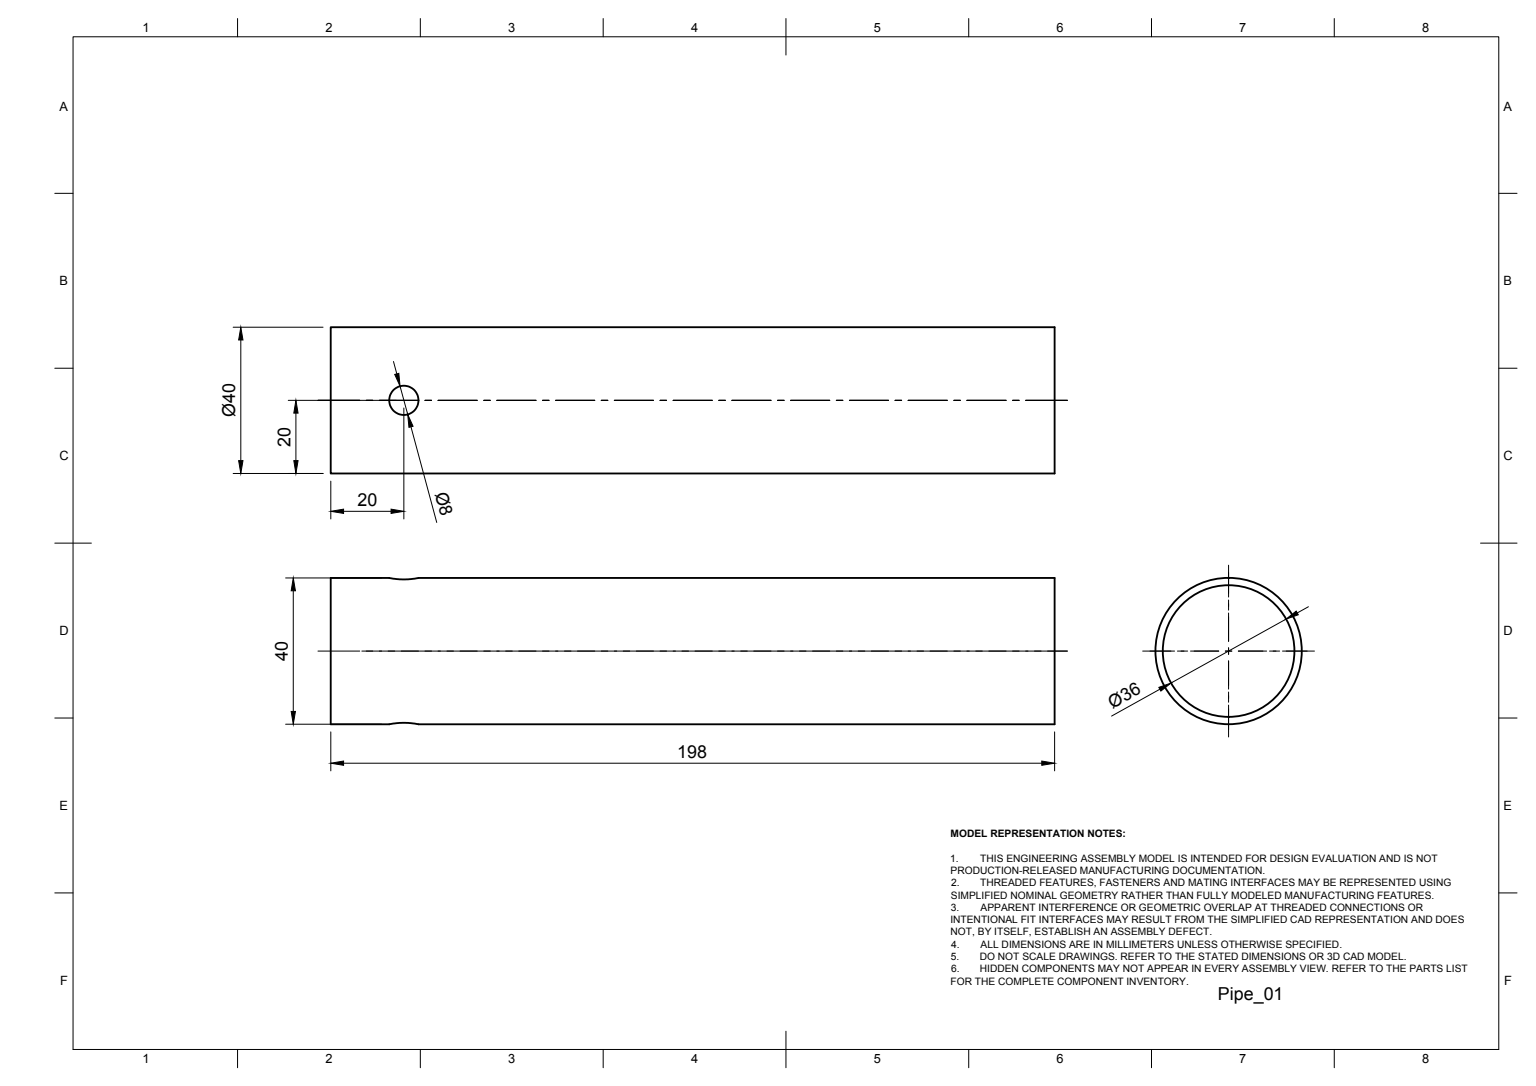
ISO-10303-21;
HEADER;
/* Generated by software containing ST-Developer
 * from STEP Tools, Inc. (www.steptools.com) 
 */

FILE_DESCRIPTION(
/* description */ (''),
/* implementation_level */ '2;1');

FILE_NAME(
/* name */ 'Pipe_01.step',
/* time_stamp */ '2026-10-06T13:31:15-07:00',
/* author */ (''),
/* organization */ (''),
/* preprocessor_version */ 'ST-DEVELOPER v20.2',
/* originating_system */ 'Autodesk Translation Framework v15.15.0.0',
/* authorisation */ '');

FILE_SCHEMA (('AUTOMOTIVE_DESIGN { 1 0 10303 214 3 1 1 }'));
ENDSEC;

DATA;
#10=MECHANICAL_DESIGN_GEOMETRIC_PRESENTATION_REPRESENTATION('',(#79),#3154);
#61=SHAPE_REPRESENTATION_RELATIONSHIP('SRR','None',#3189,#70);
#70=ADVANCED_BREP_SHAPE_REPRESENTATION('',(#88),#3145);
#79=STYLED_ITEM('',(#3243),#88);
#88=MANIFOLD_SOLID_BREP('Body1',#1081);
#97=PLANE('',#1200);
#98=PLANE('',#1201);
#128=FACE_BOUND('',#233,.T.);
#129=FACE_BOUND('',#235,.T.);
#130=FACE_BOUND('',#237,.T.);
#131=FACE_BOUND('',#239,.T.);
#139=CIRCLE('',#1195,18.);
#140=CIRCLE('',#1196,18.);
#141=CIRCLE('',#1198,20.);
#142=CIRCLE('',#1199,20.);
#171=FACE_OUTER_BOUND('',#230,.T.);
#172=FACE_OUTER_BOUND('',#231,.T.);
#173=FACE_OUTER_BOUND('',#232,.T.);
#174=FACE_OUTER_BOUND('',#234,.T.);
#175=FACE_OUTER_BOUND('',#236,.T.);
#176=FACE_OUTER_BOUND('',#238,.T.);
#230=EDGE_LOOP('',(#720,#721,#722,#723,#724,#725,#726,#727));
#231=EDGE_LOOP('',(#728,#729,#730,#731,#732,#733));
#232=EDGE_LOOP('',(#734,#735,#736,#737,#738,#739,#740,#741,#742));
#233=EDGE_LOOP('',(#743,#744));
#234=EDGE_LOOP('',(#745,#746,#747,#748,#749,#750,#751,#752,#753));
#235=EDGE_LOOP('',(#754,#755));
#236=EDGE_LOOP('',(#756));
#237=EDGE_LOOP('',(#757));
#238=EDGE_LOOP('',(#758));
#239=EDGE_LOOP('',(#759));
#300=LINE('',#1580,#366);
#301=LINE('',#1672,#367);
#302=LINE('',#1713,#368);
#303=LINE('',#1715,#369);
#304=LINE('',#1720,#370);
#305=LINE('',#1722,#371);
#366=VECTOR('',#1292,3.99999999999999);
#367=VECTOR('',#1295,3.99999999999999);
#368=VECTOR('',#1300,18.);
#369=VECTOR('',#1301,18.);
#370=VECTOR('',#1308,20.);
#371=VECTOR('',#1309,20.);
#432=B_SPLINE_CURVE_WITH_KNOTS('',3,(#1549,#1550,#1551,#1552,#1553,#1554,
#1555,#1556,#1557,#1558,#1559,#1560,#1561,#1562,#1563,#1564,#1565,#1566,
#1567),.UNSPECIFIED.,.F.,.F.,(4,2,2,2,3,2,2,2,4),(-0.604455473723513,-0.453345839217834,
-0.302236204712155,-0.151118102356077,0.,0.151118102356077,0.302236204712155,
0.453345839217834,0.604455473723513),.UNSPECIFIED.);
#433=B_SPLINE_CURVE_WITH_KNOTS('',3,(#1569,#1570,#1571,#1572,#1573,#1574,
#1575,#1576,#1577,#1578),.UNSPECIFIED.,.F.,.F.,(4,2,2,2,4),(-1.81336642117054,
-1.66225678666486,-1.51114715215918,-1.3600290498031,-1.20891094744703),
 .UNSPECIFIED.);
#434=B_SPLINE_CURVE_WITH_KNOTS('',3,(#1582,#1583,#1584,#1585,#1586,#1587,
#1588,#1589,#1590,#1591),.UNSPECIFIED.,.F.,.F.,(4,2,2,2,4),(1.20975547030872,
1.36098142054494,1.51220737078115,1.66342028812212,1.81463320546308),
 .UNSPECIFIED.);
#435=B_SPLINE_CURVE_WITH_KNOTS('',3,(#1593,#1594,#1595,#1596,#1597,#1598,
#1599,#1600,#1601,#1602,#1603,#1604,#1605,#1606,#1607,#1608,#1609,#1610,
#1611),.UNSPECIFIED.,.F.,.F.,(4,2,2,2,3,2,2,2,4),(1.81463320546308,1.96584612280404,
2.11705904014501,2.26828499038122,2.41951094061744,2.57073689085366,2.72196284108987,
2.87317575843084,3.0243886757718),.UNSPECIFIED.);
#436=B_SPLINE_CURVE_WITH_KNOTS('',3,(#1612,#1613,#1614,#1615,#1616,#1617,
#1618,#1619,#1620,#1621),.UNSPECIFIED.,.F.,.F.,(4,2,2,2,4),(0.60487773515436,
0.756090652495323,0.907303569836285,1.0585295200725,1.20975547030872),
 .UNSPECIFIED.);
#437=B_SPLINE_CURVE_WITH_KNOTS('',3,(#1622,#1623,#1624,#1625,#1626,#1627,
#1628,#1629,#1630,#1631),.UNSPECIFIED.,.F.,.F.,(4,2,2,2,4),(-1.20891094744703,
-1.05779284509095,-0.906674742734871,-0.755565108229192,-0.604455473723513),
 .UNSPECIFIED.);
#438=B_SPLINE_CURVE_WITH_KNOTS('',3,(#1635,#1636,#1637,#1638,#1639,#1640,
#1641,#1642,#1643,#1644,#1645,#1646,#1647,#1648,#1649,#1650,#1651,#1652),
 .UNSPECIFIED.,.F.,.F.,(4,2,2,2,2,2,2,2,4),(-2.41951094061744,-2.26828499038122,
-2.11705904014501,-1.96584612280404,-1.81463320546308,-1.66342028812212,
-1.51220737078115,-1.36098142054494,-1.20975547030872),.UNSPECIFIED.);
#439=B_SPLINE_CURVE_WITH_KNOTS('',3,(#1653,#1654,#1655,#1656,#1657,#1658,
#1659,#1660,#1661,#1662,#1663,#1664,#1665,#1666,#1667,#1668,#1669,#1670),
 .UNSPECIFIED.,.F.,.F.,(4,2,2,2,2,2,2,2,4),(-1.20975547030872,-1.0585295200725,
-0.907303569836286,-0.756090652495323,-0.60487773515436,-0.453664817813397,
-0.302451900472434,-0.151225950236217,0.),.UNSPECIFIED.);
#440=B_SPLINE_CURVE_WITH_KNOTS('',3,(#1674,#1675,#1676,#1677,#1678,#1679,
#1680,#1681,#1682,#1683,#1684,#1685,#1686,#1687,#1688,#1689,#1690,#1691),
 .UNSPECIFIED.,.F.,.F.,(4,2,2,2,2,2,2,2,4),(0.,0.151118102356077,0.302236204712155,
0.453345839217834,0.604455473723513,0.755565108229192,0.906674742734871,
1.05779284509095,1.20891094744703),.UNSPECIFIED.);
#441=B_SPLINE_CURVE_WITH_KNOTS('',3,(#1692,#1693,#1694,#1695,#1696,#1697,
#1698,#1699,#1700,#1701,#1702,#1703,#1704,#1705,#1706,#1707,#1708,#1709),
 .UNSPECIFIED.,.F.,.F.,(4,2,2,2,2,2,2,2,4),(1.20891094744703,1.3600290498031,
1.51114715215918,1.66225678666486,1.81336642117054,1.96447605567622,2.1155856901819,
2.26670379253797,2.41782189489405),.UNSPECIFIED.);
#478=VERTEX_POINT('',#1547);
#479=VERTEX_POINT('',#1548);
#480=VERTEX_POINT('',#1568);
#481=VERTEX_POINT('',#1579);
#482=VERTEX_POINT('',#1581);
#483=VERTEX_POINT('',#1592);
#484=VERTEX_POINT('',#1633);
#485=VERTEX_POINT('',#1634);
#486=VERTEX_POINT('',#1671);
#487=VERTEX_POINT('',#1673);
#488=VERTEX_POINT('',#1711);
#489=VERTEX_POINT('',#1714);
#490=VERTEX_POINT('',#1718);
#491=VERTEX_POINT('',#1721);
#576=EDGE_CURVE('',#478,#479,#432,.F.);
#577=EDGE_CURVE('',#480,#478,#433,.F.);
#578=EDGE_CURVE('',#480,#481,#300,.T.);
#579=EDGE_CURVE('',#482,#481,#434,.F.);
#580=EDGE_CURVE('',#483,#482,#435,.F.);
#581=EDGE_CURVE('',#481,#483,#436,.F.);
#582=EDGE_CURVE('',#479,#480,#437,.F.);
#583=EDGE_CURVE('',#484,#485,#438,.T.);
#584=EDGE_CURVE('',#485,#484,#439,.T.);
#585=EDGE_CURVE('',#485,#486,#301,.T.);
#586=EDGE_CURVE('',#487,#486,#440,.T.);
#587=EDGE_CURVE('',#486,#487,#441,.T.);
#588=EDGE_CURVE('',#488,#488,#139,.T.);
#589=EDGE_CURVE('',#488,#482,#302,.T.);
#590=EDGE_CURVE('',#483,#489,#303,.T.);
#591=EDGE_CURVE('',#489,#489,#140,.T.);
#592=EDGE_CURVE('',#490,#490,#141,.T.);
#593=EDGE_CURVE('',#490,#479,#304,.T.);
#594=EDGE_CURVE('',#478,#491,#305,.T.);
#595=EDGE_CURVE('',#491,#491,#142,.T.);
#720=ORIENTED_EDGE('',*,*,#576,.F.);
#721=ORIENTED_EDGE('',*,*,#577,.F.);
#722=ORIENTED_EDGE('',*,*,#578,.T.);
#723=ORIENTED_EDGE('',*,*,#579,.F.);
#724=ORIENTED_EDGE('',*,*,#580,.F.);
#725=ORIENTED_EDGE('',*,*,#581,.F.);
#726=ORIENTED_EDGE('',*,*,#578,.F.);
#727=ORIENTED_EDGE('',*,*,#582,.F.);
#728=ORIENTED_EDGE('',*,*,#583,.F.);
#729=ORIENTED_EDGE('',*,*,#584,.F.);
#730=ORIENTED_EDGE('',*,*,#585,.T.);
#731=ORIENTED_EDGE('',*,*,#586,.F.);
#732=ORIENTED_EDGE('',*,*,#587,.F.);
#733=ORIENTED_EDGE('',*,*,#585,.F.);
#734=ORIENTED_EDGE('',*,*,#588,.T.);
#735=ORIENTED_EDGE('',*,*,#589,.T.);
#736=ORIENTED_EDGE('',*,*,#579,.T.);
#737=ORIENTED_EDGE('',*,*,#581,.T.);
#738=ORIENTED_EDGE('',*,*,#590,.T.);
#739=ORIENTED_EDGE('',*,*,#591,.F.);
#740=ORIENTED_EDGE('',*,*,#590,.F.);
#741=ORIENTED_EDGE('',*,*,#580,.T.);
#742=ORIENTED_EDGE('',*,*,#589,.F.);
#743=ORIENTED_EDGE('',*,*,#583,.T.);
#744=ORIENTED_EDGE('',*,*,#584,.T.);
#745=ORIENTED_EDGE('',*,*,#592,.F.);
#746=ORIENTED_EDGE('',*,*,#593,.T.);
#747=ORIENTED_EDGE('',*,*,#582,.T.);
#748=ORIENTED_EDGE('',*,*,#577,.T.);
#749=ORIENTED_EDGE('',*,*,#594,.T.);
#750=ORIENTED_EDGE('',*,*,#595,.T.);
#751=ORIENTED_EDGE('',*,*,#594,.F.);
#752=ORIENTED_EDGE('',*,*,#576,.T.);
#753=ORIENTED_EDGE('',*,*,#593,.F.);
#754=ORIENTED_EDGE('',*,*,#586,.T.);
#755=ORIENTED_EDGE('',*,*,#587,.T.);
#756=ORIENTED_EDGE('',*,*,#592,.T.);
#757=ORIENTED_EDGE('',*,*,#591,.T.);
#758=ORIENTED_EDGE('',*,*,#595,.F.);
#759=ORIENTED_EDGE('',*,*,#588,.F.);
#1008=CYLINDRICAL_SURFACE('',#1192,3.99999999999999);
#1009=CYLINDRICAL_SURFACE('',#1193,3.99999999999999);
#1010=CYLINDRICAL_SURFACE('',#1194,18.);
#1011=CYLINDRICAL_SURFACE('',#1197,20.);
#1022=ADVANCED_FACE('',(#171),#1008,.F.);
#1023=ADVANCED_FACE('',(#172),#1009,.F.);
#1024=ADVANCED_FACE('',(#173,#128),#1010,.F.);
#1025=ADVANCED_FACE('',(#174,#129),#1011,.T.);
#1026=ADVANCED_FACE('',(#175,#130),#97,.T.);
#1027=ADVANCED_FACE('',(#176,#131),#98,.F.);
#1081=CLOSED_SHELL('',(#1022,#1023,#1024,#1025,#1026,#1027));
#1191=AXIS2_PLACEMENT_3D('',#1545,#1288,#1289);
#1192=AXIS2_PLACEMENT_3D('',#1546,#1290,#1291);
#1193=AXIS2_PLACEMENT_3D('',#1632,#1293,#1294);
#1194=AXIS2_PLACEMENT_3D('',#1710,#1296,#1297);
#1195=AXIS2_PLACEMENT_3D('',#1712,#1298,#1299);
#1196=AXIS2_PLACEMENT_3D('',#1716,#1302,#1303);
#1197=AXIS2_PLACEMENT_3D('',#1717,#1304,#1305);
#1198=AXIS2_PLACEMENT_3D('',#1719,#1306,#1307);
#1199=AXIS2_PLACEMENT_3D('',#1723,#1310,#1311);
#1200=AXIS2_PLACEMENT_3D('',#1724,#1312,#1313);
#1201=AXIS2_PLACEMENT_3D('',#1725,#1314,#1315);
#1288=DIRECTION('axis',(0.,0.,1.));
#1289=DIRECTION('refdir',(1.,0.,0.));
#1290=DIRECTION('center_axis',(1.,0.,0.));
#1291=DIRECTION('ref_axis',(0.,1.,0.));
#1292=DIRECTION('',(1.,0.,0.));
#1293=DIRECTION('center_axis',(1.,0.,0.));
#1294=DIRECTION('ref_axis',(0.,1.,0.));
#1295=DIRECTION('',(1.,0.,0.));
#1296=DIRECTION('center_axis',(0.,0.,1.));
#1297=DIRECTION('ref_axis',(1.,0.,0.));
#1298=DIRECTION('center_axis',(0.,0.,-1.));
#1299=DIRECTION('ref_axis',(1.,0.,0.));
#1300=DIRECTION('',(0.,0.,1.));
#1301=DIRECTION('',(0.,0.,1.));
#1302=DIRECTION('center_axis',(0.,0.,-1.));
#1303=DIRECTION('ref_axis',(1.,0.,0.));
#1304=DIRECTION('center_axis',(0.,0.,1.));
#1305=DIRECTION('ref_axis',(1.,0.,0.));
#1306=DIRECTION('center_axis',(0.,0.,1.));
#1307=DIRECTION('ref_axis',(1.,0.,0.));
#1308=DIRECTION('',(0.,0.,-1.));
#1309=DIRECTION('',(0.,0.,-1.));
#1310=DIRECTION('center_axis',(0.,0.,1.));
#1311=DIRECTION('ref_axis',(1.,0.,0.));
#1312=DIRECTION('center_axis',(0.,0.,1.));
#1313=DIRECTION('ref_axis',(1.,0.,0.));
#1314=DIRECTION('center_axis',(0.,0.,1.));
#1315=DIRECTION('ref_axis',(1.,0.,0.));
#1545=CARTESIAN_POINT('',(0.,0.,0.));
#1546=CARTESIAN_POINT('Origin',(0.,0.,180.));
#1547=CARTESIAN_POINT('',(-20.,-1.98792512857715E-15,176.));
#1548=CARTESIAN_POINT('',(-20.,-1.05117445154967E-15,184.));
#1549=CARTESIAN_POINT('Ctrl Pts',(-20.,-2.77555756156289E-16,184.));
#1550=CARTESIAN_POINT('Ctrl Pts',(-20.,0.503698781685596,184.));
#1551=CARTESIAN_POINT('Ctrl Pts',(-19.9790475458833,1.04005322432747,183.899058168943));
#1552=CARTESIAN_POINT('Ctrl Pts',(-19.9033338860745,2.02517944479051,183.490417366179));
#1553=CARTESIAN_POINT('Ctrl Pts',(-19.8496135055327,2.47406169858037,183.182792550912));
#1554=CARTESIAN_POINT('Ctrl Pts',(-19.7483634040773,3.18281240876835,182.474041840724));
#1555=CARTESIAN_POINT('Ctrl Pts',(-19.6941660317108,3.4904216705935,182.02516802012));
#1556=CARTESIAN_POINT('Ctrl Pts',(-19.6173550647379,3.89905118499443,181.040071108648));
#1557=CARTESIAN_POINT('Ctrl Pts',(-19.5959179422654,3.99999999999999,180.503727007854));
#1558=CARTESIAN_POINT('Ctrl Pts',(-19.5959179422654,3.99999999999999,180.));
#1559=CARTESIAN_POINT('Ctrl Pts',(-19.5959179422654,3.99999999999999,179.496272992146));
#1560=CARTESIAN_POINT('Ctrl Pts',(-19.6173550647379,3.89905118499443,178.959928891352));
#1561=CARTESIAN_POINT('Ctrl Pts',(-19.6941660317108,3.4904216705935,177.97483197988));
#1562=CARTESIAN_POINT('Ctrl Pts',(-19.7483634040773,3.18281240876835,177.525958159276));
#1563=CARTESIAN_POINT('Ctrl Pts',(-19.8496135055327,2.47406169858037,176.817207449088));
#1564=CARTESIAN_POINT('Ctrl Pts',(-19.9033338860745,2.02517944479051,176.509582633821));
#1565=CARTESIAN_POINT('Ctrl Pts',(-19.9790475458833,1.04005322432747,176.100941831057));
#1566=CARTESIAN_POINT('Ctrl Pts',(-20.,0.503698781685596,176.));
#1567=CARTESIAN_POINT('Ctrl Pts',(-20.,-1.2490009027033E-15,176.));
#1568=CARTESIAN_POINT('',(-19.5959179422654,-3.99999999999999,180.));
#1569=CARTESIAN_POINT('Ctrl Pts',(-20.,-9.71445146547012E-16,176.));
#1570=CARTESIAN_POINT('Ctrl Pts',(-20.,-0.503698781685598,176.));
#1571=CARTESIAN_POINT('Ctrl Pts',(-19.9790475458833,-1.04005322432746,176.100941831057));
#1572=CARTESIAN_POINT('Ctrl Pts',(-19.9033338860745,-2.0251794447905,176.509582633821));
#1573=CARTESIAN_POINT('Ctrl Pts',(-19.8496135055327,-2.47406169858037,176.817207449088));
#1574=CARTESIAN_POINT('Ctrl Pts',(-19.7483634040773,-3.18281240876835,177.525958159276));
#1575=CARTESIAN_POINT('Ctrl Pts',(-19.6941660317108,-3.4904216705935,177.97483197988));
#1576=CARTESIAN_POINT('Ctrl Pts',(-19.6173550647379,-3.89905118499443,178.959928891352));
#1577=CARTESIAN_POINT('Ctrl Pts',(-19.5959179422654,-3.99999999999999,179.496272992146));
#1578=CARTESIAN_POINT('Ctrl Pts',(-19.5959179422654,-3.99999999999999,180.));
#1579=CARTESIAN_POINT('',(-17.5499287747842,-3.99999999999999,180.));
#1580=CARTESIAN_POINT('',(0.,-3.99999999999999,180.));
#1581=CARTESIAN_POINT('',(-18.,-2.48996090001406E-15,176.));
#1582=CARTESIAN_POINT('Ctrl Pts',(-17.5499287747842,-3.99999999999999,180.));
#1583=CARTESIAN_POINT('Ctrl Pts',(-17.5499287747842,-3.99999999999999,179.495913499213));
#1584=CARTESIAN_POINT('Ctrl Pts',(-17.5739034455062,-3.89891257329756,178.959425202916));
#1585=CARTESIAN_POINT('Ctrl Pts',(-17.6596205619409,-3.49018656101197,177.97443488127));
#1586=CARTESIAN_POINT('Ctrl Pts',(-17.7200302505161,-3.18263533348267,177.52578108399));
#1587=CARTESIAN_POINT('Ctrl Pts',(-17.8327425616729,-2.47424944224197,176.81739519275));
#1588=CARTESIAN_POINT('Ctrl Pts',(-17.8924945311419,-2.02558278587652,176.509820096788));
#1589=CARTESIAN_POINT('Ctrl Pts',(-17.9766962279685,-1.04054739507664,176.101076729386));
#1590=CARTESIAN_POINT('Ctrl Pts',(-18.,-0.504043057803209,176.));
#1591=CARTESIAN_POINT('Ctrl Pts',(-18.,9.71445146547012E-16,176.));
#1592=CARTESIAN_POINT('',(-18.,-2.28179408289685E-15,184.));
#1593=CARTESIAN_POINT('Ctrl Pts',(-18.,-2.77555756156289E-15,176.));
#1594=CARTESIAN_POINT('Ctrl Pts',(-18.,0.504043057803207,176.));
#1595=CARTESIAN_POINT('Ctrl Pts',(-17.9766962279685,1.04054739507664,176.101076729386));
#1596=CARTESIAN_POINT('Ctrl Pts',(-17.8924945311419,2.02558278587652,176.509820096788));
#1597=CARTESIAN_POINT('Ctrl Pts',(-17.8327425616729,2.47424944224197,176.81739519275));
#1598=CARTESIAN_POINT('Ctrl Pts',(-17.7200302505161,3.18263533348267,177.52578108399));
#1599=CARTESIAN_POINT('Ctrl Pts',(-17.6596205619409,3.49018656101197,177.97443488127));
#1600=CARTESIAN_POINT('Ctrl Pts',(-17.5739034455062,3.89891257329756,178.959425202916));
#1601=CARTESIAN_POINT('Ctrl Pts',(-17.5499287747842,3.99999999999999,179.495913499213));
#1602=CARTESIAN_POINT('Ctrl Pts',(-17.5499287747842,3.99999999999999,180.));
#1603=CARTESIAN_POINT('Ctrl Pts',(-17.5499287747842,3.99999999999999,180.504086500787));
#1604=CARTESIAN_POINT('Ctrl Pts',(-17.5739034455062,3.89891257329756,181.040574797084));
#1605=CARTESIAN_POINT('Ctrl Pts',(-17.6596205619409,3.49018656101197,182.02556511873));
#1606=CARTESIAN_POINT('Ctrl Pts',(-17.7200302505161,3.18263533348267,182.47421891601));
#1607=CARTESIAN_POINT('Ctrl Pts',(-17.8327425616729,2.47424944224197,183.18260480725));
#1608=CARTESIAN_POINT('Ctrl Pts',(-17.8924945311419,2.02558278587652,183.490179903212));
#1609=CARTESIAN_POINT('Ctrl Pts',(-17.9766962279685,1.04054739507664,183.898923270614));
#1610=CARTESIAN_POINT('Ctrl Pts',(-18.,0.50404305780321,184.));
#1611=CARTESIAN_POINT('Ctrl Pts',(-18.,6.93889390390723E-16,184.));
#1612=CARTESIAN_POINT('Ctrl Pts',(-18.,7.63278329429795E-16,184.));
#1613=CARTESIAN_POINT('Ctrl Pts',(-18.,-0.504043057803209,184.));
#1614=CARTESIAN_POINT('Ctrl Pts',(-17.9766962279685,-1.04054739507664,183.898923270614));
#1615=CARTESIAN_POINT('Ctrl Pts',(-17.8924945311419,-2.02558278587652,183.490179903212));
#1616=CARTESIAN_POINT('Ctrl Pts',(-17.8327425616729,-2.47424944224197,183.18260480725));
#1617=CARTESIAN_POINT('Ctrl Pts',(-17.7200302505161,-3.18263533348267,182.47421891601));
#1618=CARTESIAN_POINT('Ctrl Pts',(-17.6596205619409,-3.49018656101197,182.02556511873));
#1619=CARTESIAN_POINT('Ctrl Pts',(-17.5739034455062,-3.89891257329756,181.040574797084));
#1620=CARTESIAN_POINT('Ctrl Pts',(-17.5499287747842,-3.99999999999999,180.504086500787));
#1621=CARTESIAN_POINT('Ctrl Pts',(-17.5499287747842,-3.99999999999999,180.));
#1622=CARTESIAN_POINT('Ctrl Pts',(-19.5959179422654,-3.99999999999999,180.));
#1623=CARTESIAN_POINT('Ctrl Pts',(-19.5959179422654,-3.99999999999999,180.503727007854));
#1624=CARTESIAN_POINT('Ctrl Pts',(-19.6173550647379,-3.89905118499443,181.040071108648));
#1625=CARTESIAN_POINT('Ctrl Pts',(-19.6941660317108,-3.4904216705935,182.02516802012));
#1626=CARTESIAN_POINT('Ctrl Pts',(-19.7483634040773,-3.18281240876835,182.474041840724));
#1627=CARTESIAN_POINT('Ctrl Pts',(-19.8496135055327,-2.47406169858037,183.182792550912));
#1628=CARTESIAN_POINT('Ctrl Pts',(-19.9033338860745,-2.02517944479051,183.490417366179));
#1629=CARTESIAN_POINT('Ctrl Pts',(-19.9790475458833,-1.04005322432747,183.899058168943));
#1630=CARTESIAN_POINT('Ctrl Pts',(-20.,-0.503698781685596,184.));
#1631=CARTESIAN_POINT('Ctrl Pts',(-20.,3.46944695195361E-16,184.));
#1632=CARTESIAN_POINT('Origin',(0.,0.,180.));
#1633=CARTESIAN_POINT('',(17.5499287747842,3.99999999999999,180.));
#1634=CARTESIAN_POINT('',(17.5499287747842,-3.99999999999999,180.));
#1635=CARTESIAN_POINT('Ctrl Pts',(17.5499287747842,3.99999999999999,180.));
#1636=CARTESIAN_POINT('Ctrl Pts',(17.5499287747842,3.99999999999999,180.504086500787));
#1637=CARTESIAN_POINT('Ctrl Pts',(17.5739034455062,3.89891257329756,181.040574797084));
#1638=CARTESIAN_POINT('Ctrl Pts',(17.6596205619409,3.49018656101197,182.02556511873));
#1639=CARTESIAN_POINT('Ctrl Pts',(17.7200302505161,3.18263533348267,182.47421891601));
#1640=CARTESIAN_POINT('Ctrl Pts',(17.8327425616729,2.47424944224197,183.18260480725));
#1641=CARTESIAN_POINT('Ctrl Pts',(17.8924945311419,2.0255827858765,183.490179903212));
#1642=CARTESIAN_POINT('Ctrl Pts',(17.9766962279685,1.04054739507661,183.898923270614));
#1643=CARTESIAN_POINT('Ctrl Pts',(18.,0.50404305780321,184.));
#1644=CARTESIAN_POINT('Ctrl Pts',(18.,-0.504043057803209,184.));
#1645=CARTESIAN_POINT('Ctrl Pts',(17.9766962279685,-1.04054739507664,183.898923270614));
#1646=CARTESIAN_POINT('Ctrl Pts',(17.8924945311419,-2.02558278587652,183.490179903212));
#1647=CARTESIAN_POINT('Ctrl Pts',(17.8327425616729,-2.47424944224197,183.18260480725));
#1648=CARTESIAN_POINT('Ctrl Pts',(17.7200302505161,-3.18263533348267,182.47421891601));
#1649=CARTESIAN_POINT('Ctrl Pts',(17.6596205619409,-3.49018656101197,182.02556511873));
#1650=CARTESIAN_POINT('Ctrl Pts',(17.5739034455062,-3.89891257329756,181.040574797084));
#1651=CARTESIAN_POINT('Ctrl Pts',(17.5499287747842,-3.99999999999999,180.504086500787));
#1652=CARTESIAN_POINT('Ctrl Pts',(17.5499287747842,-3.99999999999999,180.));
#1653=CARTESIAN_POINT('Ctrl Pts',(17.5499287747842,-3.99999999999999,180.));
#1654=CARTESIAN_POINT('Ctrl Pts',(17.5499287747842,-3.99999999999999,179.495913499213));
#1655=CARTESIAN_POINT('Ctrl Pts',(17.5739034455062,-3.89891257329756,178.959425202916));
#1656=CARTESIAN_POINT('Ctrl Pts',(17.6596205619409,-3.49018656101197,177.97443488127));
#1657=CARTESIAN_POINT('Ctrl Pts',(17.7200302505161,-3.18263533348267,177.52578108399));
#1658=CARTESIAN_POINT('Ctrl Pts',(17.8327425616729,-2.47424944224197,176.81739519275));
#1659=CARTESIAN_POINT('Ctrl Pts',(17.8924945311419,-2.02558278587652,176.509820096788));
#1660=CARTESIAN_POINT('Ctrl Pts',(17.9766962279685,-1.04054739507664,176.101076729386));
#1661=CARTESIAN_POINT('Ctrl Pts',(18.,-0.50404305780321,176.));
#1662=CARTESIAN_POINT('Ctrl Pts',(18.,0.504043057803209,176.));
#1663=CARTESIAN_POINT('Ctrl Pts',(17.9766962279685,1.04054739507664,176.101076729386));
#1664=CARTESIAN_POINT('Ctrl Pts',(17.8924945311419,2.02558278587652,176.509820096788));
#1665=CARTESIAN_POINT('Ctrl Pts',(17.8327425616729,2.47424944224197,176.81739519275));
#1666=CARTESIAN_POINT('Ctrl Pts',(17.7200302505161,3.18263533348267,177.52578108399));
#1667=CARTESIAN_POINT('Ctrl Pts',(17.6596205619409,3.49018656101197,177.97443488127));
#1668=CARTESIAN_POINT('Ctrl Pts',(17.5739034455062,3.89891257329756,178.959425202916));
#1669=CARTESIAN_POINT('Ctrl Pts',(17.5499287747842,3.99999999999999,179.495913499213));
#1670=CARTESIAN_POINT('Ctrl Pts',(17.5499287747842,3.99999999999999,180.));
#1671=CARTESIAN_POINT('',(19.5959179422654,-3.99999999999999,180.));
#1672=CARTESIAN_POINT('',(0.,-3.99999999999999,180.));
#1673=CARTESIAN_POINT('',(19.5959179422654,3.99999999999999,180.));
#1674=CARTESIAN_POINT('Ctrl Pts',(19.5959179422654,3.99999999999999,180.));
#1675=CARTESIAN_POINT('Ctrl Pts',(19.5959179422654,3.99999999999999,179.496272992146));
#1676=CARTESIAN_POINT('Ctrl Pts',(19.6173550647379,3.89905118499443,178.959928891352));
#1677=CARTESIAN_POINT('Ctrl Pts',(19.6941660317108,3.4904216705935,177.97483197988));
#1678=CARTESIAN_POINT('Ctrl Pts',(19.7483634040773,3.18281240876835,177.525958159276));
#1679=CARTESIAN_POINT('Ctrl Pts',(19.8496135055327,2.47406169858037,176.817207449088));
#1680=CARTESIAN_POINT('Ctrl Pts',(19.9033338860745,2.02517944479051,176.509582633821));
#1681=CARTESIAN_POINT('Ctrl Pts',(19.9790475458833,1.04005322432747,176.100941831057));
#1682=CARTESIAN_POINT('Ctrl Pts',(20.,0.503698781685596,176.));
#1683=CARTESIAN_POINT('Ctrl Pts',(20.,-0.503698781685597,176.));
#1684=CARTESIAN_POINT('Ctrl Pts',(19.9790475458833,-1.04005322432747,176.100941831057));
#1685=CARTESIAN_POINT('Ctrl Pts',(19.9033338860745,-2.02517944479051,176.509582633821));
#1686=CARTESIAN_POINT('Ctrl Pts',(19.8496135055327,-2.47406169858037,176.817207449088));
#1687=CARTESIAN_POINT('Ctrl Pts',(19.7483634040773,-3.18281240876835,177.525958159276));
#1688=CARTESIAN_POINT('Ctrl Pts',(19.6941660317108,-3.4904216705935,177.97483197988));
#1689=CARTESIAN_POINT('Ctrl Pts',(19.6173550647379,-3.89905118499443,178.959928891352));
#1690=CARTESIAN_POINT('Ctrl Pts',(19.5959179422654,-3.99999999999999,179.496272992146));
#1691=CARTESIAN_POINT('Ctrl Pts',(19.5959179422654,-3.99999999999999,180.));
#1692=CARTESIAN_POINT('Ctrl Pts',(19.5959179422654,-3.99999999999999,180.));
#1693=CARTESIAN_POINT('Ctrl Pts',(19.5959179422654,-3.99999999999999,180.503727007854));
#1694=CARTESIAN_POINT('Ctrl Pts',(19.6173550647379,-3.89905118499443,181.040071108648));
#1695=CARTESIAN_POINT('Ctrl Pts',(19.6941660317108,-3.49042167059349,182.02516802012));
#1696=CARTESIAN_POINT('Ctrl Pts',(19.7483634040773,-3.18281240876835,182.474041840724));
#1697=CARTESIAN_POINT('Ctrl Pts',(19.8496135055327,-2.47406169858037,183.182792550912));
#1698=CARTESIAN_POINT('Ctrl Pts',(19.9033338860745,-2.02517944479048,183.490417366179));
#1699=CARTESIAN_POINT('Ctrl Pts',(19.9790475458833,-1.04005322432745,183.899058168943));
#1700=CARTESIAN_POINT('Ctrl Pts',(20.,-0.503698781685597,184.));
#1701=CARTESIAN_POINT('Ctrl Pts',(20.,0.503698781685597,184.));
#1702=CARTESIAN_POINT('Ctrl Pts',(19.9790475458833,1.04005322432747,183.899058168943));
#1703=CARTESIAN_POINT('Ctrl Pts',(19.9033338860745,2.02517944479051,183.490417366179));
#1704=CARTESIAN_POINT('Ctrl Pts',(19.8496135055327,2.47406169858037,183.182792550912));
#1705=CARTESIAN_POINT('Ctrl Pts',(19.7483634040773,3.18281240876835,182.474041840724));
#1706=CARTESIAN_POINT('Ctrl Pts',(19.6941660317108,3.4904216705935,182.02516802012));
#1707=CARTESIAN_POINT('Ctrl Pts',(19.6173550647379,3.89905118499443,181.040071108648));
#1708=CARTESIAN_POINT('Ctrl Pts',(19.5959179422654,3.99999999999999,180.503727007854));
#1709=CARTESIAN_POINT('Ctrl Pts',(19.5959179422654,3.99999999999999,180.));
#1710=CARTESIAN_POINT('Origin',(0.,0.,0.));
#1711=CARTESIAN_POINT('',(-18.,2.20436423846524E-15,2.));
#1712=CARTESIAN_POINT('Origin',(0.,0.,2.));
#1713=CARTESIAN_POINT('',(-18.,-2.20436423846524E-15,0.));
#1714=CARTESIAN_POINT('',(-18.,-2.20436423846524E-15,200.));
#1715=CARTESIAN_POINT('',(-18.,-2.20436423846524E-15,0.));
#1716=CARTESIAN_POINT('Origin',(0.,0.,200.));
#1717=CARTESIAN_POINT('Origin',(0.,0.,0.));
#1718=CARTESIAN_POINT('',(-20.,-2.44929359829471E-15,200.));
#1719=CARTESIAN_POINT('Origin',(0.,0.,200.));
#1720=CARTESIAN_POINT('',(-20.,-2.44929359829471E-15,0.));
#1721=CARTESIAN_POINT('',(-20.,-2.44929359829471E-15,2.));
#1722=CARTESIAN_POINT('',(-20.,-2.44929359829471E-15,0.));
#1723=CARTESIAN_POINT('Origin',(0.,0.,2.));
#1724=CARTESIAN_POINT('Origin',(0.,0.,200.));
#1725=CARTESIAN_POINT('Origin',(0.,0.,2.));
#3134=UNCERTAINTY_MEASURE_WITH_UNIT(LENGTH_MEASURE(0.01),#3155,
'DISTANCE_ACCURACY_VALUE',
'Maximum model space distance between geometric entities at asserted c
onnectivities');
#3143=UNCERTAINTY_MEASURE_WITH_UNIT(LENGTH_MEASURE(0.01),#3155,
'DISTANCE_ACCURACY_VALUE',
'Maximum model space distance between geometric entities at asserted c
onnectivities');
#3145=(
GEOMETRIC_REPRESENTATION_CONTEXT(3)
GLOBAL_UNCERTAINTY_ASSIGNED_CONTEXT((#3134))
GLOBAL_UNIT_ASSIGNED_CONTEXT((#3155,#3157,#3158))
REPRESENTATION_CONTEXT('','3D')
);
#3154=(
GEOMETRIC_REPRESENTATION_CONTEXT(3)
GLOBAL_UNCERTAINTY_ASSIGNED_CONTEXT((#3143))
GLOBAL_UNIT_ASSIGNED_CONTEXT((#3155,#3157,#3158))
REPRESENTATION_CONTEXT('','3D')
);
#3155=(
LENGTH_UNIT()
NAMED_UNIT(*)
SI_UNIT(.MILLI.,.METRE.)
);
#3157=(
NAMED_UNIT(*)
PLANE_ANGLE_UNIT()
SI_UNIT($,.RADIAN.)
);
#3158=(
NAMED_UNIT(*)
SI_UNIT($,.STERADIAN.)
SOLID_ANGLE_UNIT()
);
#3160=SHAPE_DEFINITION_REPRESENTATION(#3170,#3189);
#3170=PRODUCT_DEFINITION_SHAPE('',$,#3200);
#3189=SHAPE_REPRESENTATION('',(#1191),#3145);
#3198=PRODUCT_DEFINITION_CONTEXT('part definition',#3230,'design');
#3200=PRODUCT_DEFINITION('Pipe_01','Pipe_01',#3210,#3198);
#3210=PRODUCT_DEFINITION_FORMATION('',$,#3233);
#3230=APPLICATION_CONTEXT(
'Core Data for Automotive Mechanical Design Process');
#3231=PRODUCT_CONTEXT('part definition',#3230,'mechanical');
#3233=PRODUCT('Pipe_01','Pipe_01',$,(#3231));
#3243=PRESENTATION_STYLE_ASSIGNMENT((#3245));
#3245=SURFACE_STYLE_USAGE(.BOTH.,#3247);
#3247=SURFACE_SIDE_STYLE('',(#3249));
#3249=SURFACE_STYLE_FILL_AREA(#3251);
#3251=FILL_AREA_STYLE('Opaque(160,160,160)',(#3253));
#3253=FILL_AREA_STYLE_COLOUR('Opaque(160,160,160)',#3255);
#3255=COLOUR_RGB('Opaque(160,160,160)', 0.09019608, 0.27058824, 0.51372549);
ENDSEC;
END-ISO-10303-21;
